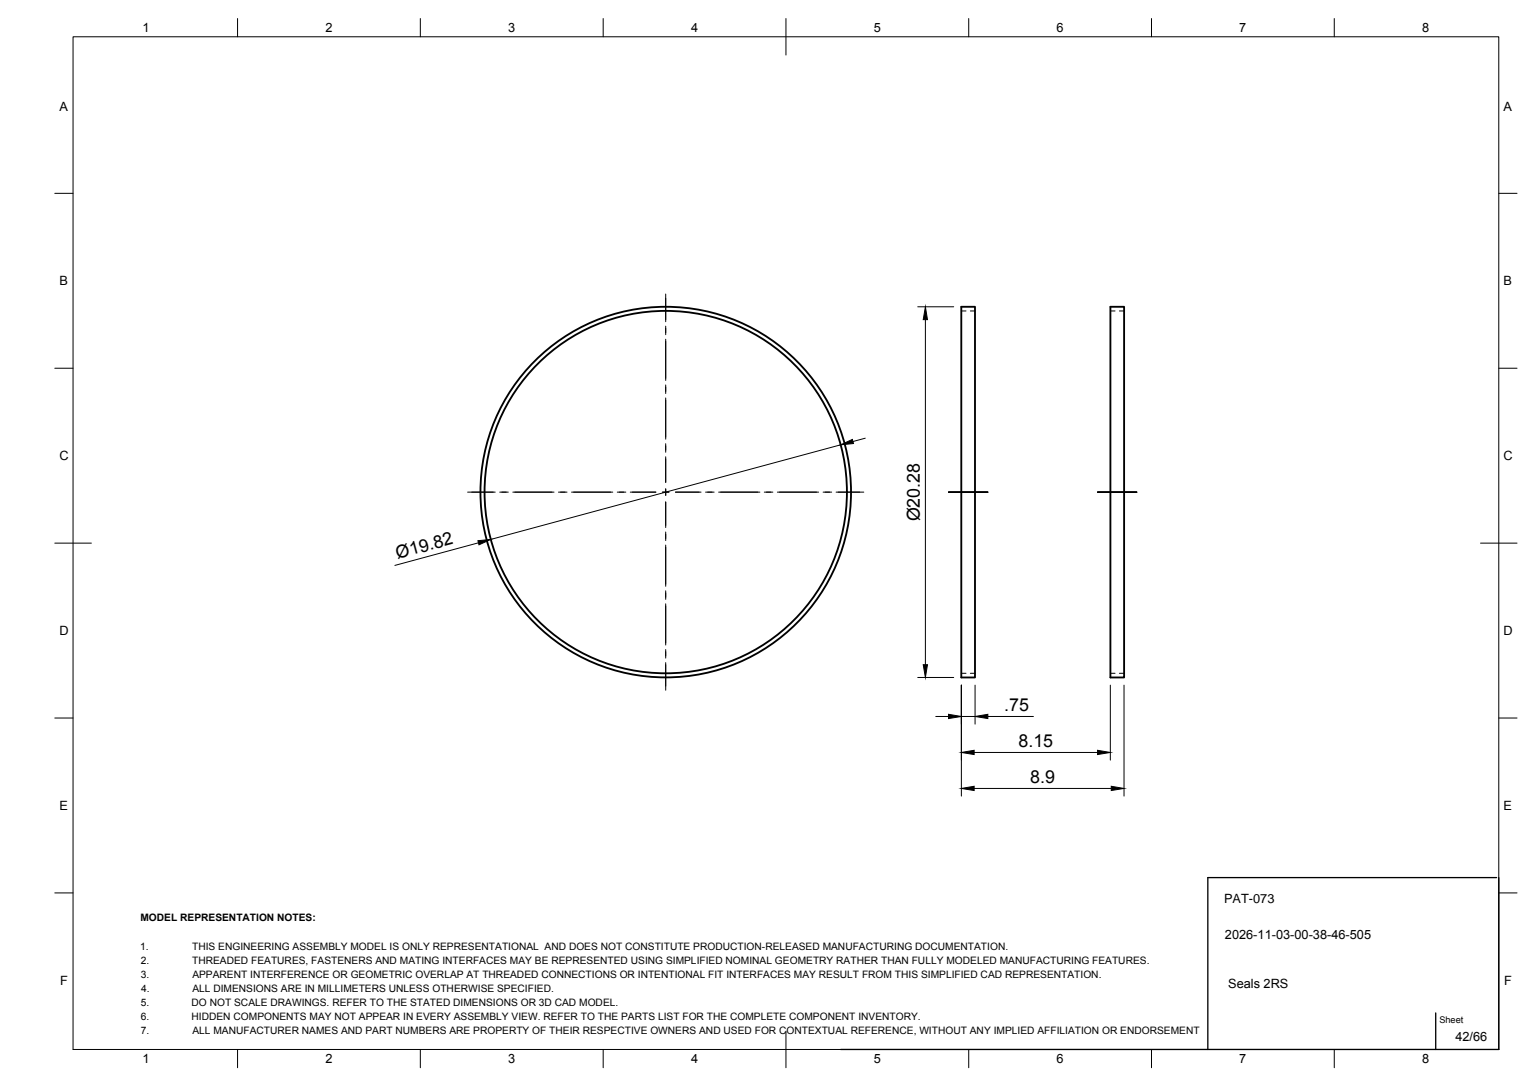
ISO-10303-21;
HEADER;
/* Generated by software containing ST-Developer
 * from STEP Tools, Inc. (www.steptools.com) 
 */

FILE_DESCRIPTION(
/* description */ ('Manual piston pump'),
/* implementation_level */ '2;1');

FILE_NAME(
/* name */ 'Seals 2RS.step',
/* time_stamp */ '2026-11-02T16:54:23-08:00',
/* author */ (''),
/* organization */ (''),
/* preprocessor_version */ 'ST-DEVELOPER v20.2',
/* originating_system */ 'Autodesk Translation Framework v15.17.0.0',
/* authorisation */ '');

FILE_SCHEMA (('AUTOMOTIVE_DESIGN { 1 0 10303 214 3 1 1 }'));
ENDSEC;

DATA;
#10=MECHANICAL_DESIGN_GEOMETRIC_PRESENTATION_REPRESENTATION('',(#722,#723),#19043);
#589=SHAPE_REPRESENTATION_RELATIONSHIP('SRR','None',#19336,#652);
#652=ADVANCED_BREP_SHAPE_REPRESENTATION('',(#792,#793),#19003);
#722=STYLED_ITEM('',(#19661),#792);
#723=STYLED_ITEM('',(#19661),#793);
#792=MANIFOLD_SOLID_BREP('Body1',#9508);
#793=MANIFOLD_SOLID_BREP('Body2',#9509);
#951=FACE_BOUND('',#2273,.T.);
#952=FACE_BOUND('',#2276,.T.);
#953=FACE_BOUND('',#2279,.T.);
#954=FACE_BOUND('',#2282,.T.);
#1191=CYLINDRICAL_SURFACE('',#10820,1.013815);
#1192=CYLINDRICAL_SURFACE('',#10824,0.991185);
#1193=CYLINDRICAL_SURFACE('',#10828,1.013815);
#1194=CYLINDRICAL_SURFACE('',#10832,0.991185);
#1573=FACE_OUTER_BOUND('',#2272,.T.);
#1574=FACE_OUTER_BOUND('',#2274,.T.);
#1575=FACE_OUTER_BOUND('',#2275,.T.);
#1576=FACE_OUTER_BOUND('',#2277,.T.);
#1577=FACE_OUTER_BOUND('',#2278,.T.);
#1578=FACE_OUTER_BOUND('',#2280,.T.);
#1579=FACE_OUTER_BOUND('',#2281,.T.);
#1580=FACE_OUTER_BOUND('',#2283,.T.);
#2272=EDGE_LOOP('',(#7437));
#2273=EDGE_LOOP('',(#7438));
#2274=EDGE_LOOP('',(#7439,#7440,#7441,#7442));
#2275=EDGE_LOOP('',(#7443));
#2276=EDGE_LOOP('',(#7444));
#2277=EDGE_LOOP('',(#7445,#7446,#7447,#7448));
#2278=EDGE_LOOP('',(#7449));
#2279=EDGE_LOOP('',(#7450));
#2280=EDGE_LOOP('',(#7451,#7452,#7453,#7454));
#2281=EDGE_LOOP('',(#7455));
#2282=EDGE_LOOP('',(#7456));
#2283=EDGE_LOOP('',(#7457,#7458,#7459,#7460));
#2925=CIRCLE('',#10818,1.013815);
#2926=CIRCLE('',#10819,0.991185);
#2927=CIRCLE('',#10821,1.013815);
#2928=CIRCLE('',#10823,0.991185);
#2929=CIRCLE('',#10826,1.013815);
#2930=CIRCLE('',#10827,0.991185);
#2931=CIRCLE('',#10829,1.013815);
#2932=CIRCLE('',#10831,0.991185);
#3434=LINE('',#16311,#4038);
#3435=LINE('',#16316,#4039);
#3436=LINE('',#16325,#4040);
#3437=LINE('',#16330,#4041);
#4038=VECTOR('',#12940,1.013815);
#4039=VECTOR('',#12947,0.991185);
#4040=VECTOR('',#12958,1.013815);
#4041=VECTOR('',#12965,0.991185);
#4748=VERTEX_POINT('',#16304);
#4749=VERTEX_POINT('',#16306);
#4750=VERTEX_POINT('',#16309);
#4751=VERTEX_POINT('',#16313);
#4752=VERTEX_POINT('',#16318);
#4753=VERTEX_POINT('',#16320);
#4754=VERTEX_POINT('',#16323);
#4755=VERTEX_POINT('',#16327);
#5705=EDGE_CURVE('',#4748,#4748,#2925,.T.);
#5706=EDGE_CURVE('',#4749,#4749,#2926,.T.);
#5707=EDGE_CURVE('',#4750,#4750,#2927,.T.);
#5708=EDGE_CURVE('',#4750,#4748,#3434,.T.);
#5709=EDGE_CURVE('',#4751,#4751,#2928,.T.);
#5710=EDGE_CURVE('',#4751,#4749,#3435,.T.);
#5711=EDGE_CURVE('',#4752,#4752,#2929,.T.);
#5712=EDGE_CURVE('',#4753,#4753,#2930,.T.);
#5713=EDGE_CURVE('',#4754,#4754,#2931,.T.);
#5714=EDGE_CURVE('',#4754,#4752,#3436,.T.);
#5715=EDGE_CURVE('',#4755,#4755,#2932,.T.);
#5716=EDGE_CURVE('',#4755,#4753,#3437,.T.);
#7437=ORIENTED_EDGE('',*,*,#5705,.F.);
#7438=ORIENTED_EDGE('',*,*,#5706,.T.);
#7439=ORIENTED_EDGE('',*,*,#5707,.F.);
#7440=ORIENTED_EDGE('',*,*,#5708,.T.);
#7441=ORIENTED_EDGE('',*,*,#5705,.T.);
#7442=ORIENTED_EDGE('',*,*,#5708,.F.);
#7443=ORIENTED_EDGE('',*,*,#5707,.T.);
#7444=ORIENTED_EDGE('',*,*,#5709,.F.);
#7445=ORIENTED_EDGE('',*,*,#5709,.T.);
#7446=ORIENTED_EDGE('',*,*,#5710,.T.);
#7447=ORIENTED_EDGE('',*,*,#5706,.F.);
#7448=ORIENTED_EDGE('',*,*,#5710,.F.);
#7449=ORIENTED_EDGE('',*,*,#5711,.F.);
#7450=ORIENTED_EDGE('',*,*,#5712,.T.);
#7451=ORIENTED_EDGE('',*,*,#5713,.F.);
#7452=ORIENTED_EDGE('',*,*,#5714,.T.);
#7453=ORIENTED_EDGE('',*,*,#5711,.T.);
#7454=ORIENTED_EDGE('',*,*,#5714,.F.);
#7455=ORIENTED_EDGE('',*,*,#5713,.T.);
#7456=ORIENTED_EDGE('',*,*,#5715,.F.);
#7457=ORIENTED_EDGE('',*,*,#5715,.T.);
#7458=ORIENTED_EDGE('',*,*,#5716,.T.);
#7459=ORIENTED_EDGE('',*,*,#5712,.F.);
#7460=ORIENTED_EDGE('',*,*,#5716,.F.);
#8721=PLANE('',#10817);
#8722=PLANE('',#10822);
#8723=PLANE('',#10825);
#8724=PLANE('',#10830);
#9178=ADVANCED_FACE('',(#1573,#951),#8721,.T.);
#9179=ADVANCED_FACE('',(#1574),#1191,.T.);
#9180=ADVANCED_FACE('',(#1575,#952),#8722,.T.);
#9181=ADVANCED_FACE('',(#1576),#1192,.F.);
#9182=ADVANCED_FACE('',(#1577,#953),#8723,.T.);
#9183=ADVANCED_FACE('',(#1578),#1193,.T.);
#9184=ADVANCED_FACE('',(#1579,#954),#8724,.T.);
#9185=ADVANCED_FACE('',(#1580),#1194,.F.);
#9508=CLOSED_SHELL('',(#9178,#9179,#9180,#9181));
#9509=CLOSED_SHELL('',(#9182,#9183,#9184,#9185));
#10816=AXIS2_PLACEMENT_3D('',#16302,#12928,#12929);
#10817=AXIS2_PLACEMENT_3D('',#16303,#12930,#12931);
#10818=AXIS2_PLACEMENT_3D('',#16305,#12932,#12933);
#10819=AXIS2_PLACEMENT_3D('',#16307,#12934,#12935);
#10820=AXIS2_PLACEMENT_3D('',#16308,#12936,#12937);
#10821=AXIS2_PLACEMENT_3D('',#16310,#12938,#12939);
#10822=AXIS2_PLACEMENT_3D('',#16312,#12941,#12942);
#10823=AXIS2_PLACEMENT_3D('',#16314,#12943,#12944);
#10824=AXIS2_PLACEMENT_3D('',#16315,#12945,#12946);
#10825=AXIS2_PLACEMENT_3D('',#16317,#12948,#12949);
#10826=AXIS2_PLACEMENT_3D('',#16319,#12950,#12951);
#10827=AXIS2_PLACEMENT_3D('',#16321,#12952,#12953);
#10828=AXIS2_PLACEMENT_3D('',#16322,#12954,#12955);
#10829=AXIS2_PLACEMENT_3D('',#16324,#12956,#12957);
#10830=AXIS2_PLACEMENT_3D('',#16326,#12959,#12960);
#10831=AXIS2_PLACEMENT_3D('',#16328,#12961,#12962);
#10832=AXIS2_PLACEMENT_3D('',#16329,#12963,#12964);
#12928=DIRECTION('axis',(0.,0.,1.));
#12929=DIRECTION('refdir',(1.,0.,0.));
#12930=DIRECTION('center_axis',(0.,1.,0.));
#12931=DIRECTION('ref_axis',(0.,0.,1.));
#12932=DIRECTION('center_axis',(0.,-1.,0.));
#12933=DIRECTION('ref_axis',(1.,0.,0.));
#12934=DIRECTION('center_axis',(0.,-1.,0.));
#12935=DIRECTION('ref_axis',(1.,0.,0.));
#12936=DIRECTION('center_axis',(0.,-1.,0.));
#12937=DIRECTION('ref_axis',(1.,0.,0.));
#12938=DIRECTION('center_axis',(0.,-1.,0.));
#12939=DIRECTION('ref_axis',(1.,0.,0.));
#12940=DIRECTION('',(0.,1.,0.));
#12941=DIRECTION('center_axis',(0.,-1.,0.));
#12942=DIRECTION('ref_axis',(0.,0.,-1.));
#12943=DIRECTION('center_axis',(0.,-1.,0.));
#12944=DIRECTION('ref_axis',(1.,0.,0.));
#12945=DIRECTION('center_axis',(0.,-1.,0.));
#12946=DIRECTION('ref_axis',(1.,0.,0.));
#12947=DIRECTION('',(0.,1.,0.));
#12948=DIRECTION('center_axis',(0.,1.,0.));
#12949=DIRECTION('ref_axis',(0.,0.,1.));
#12950=DIRECTION('center_axis',(0.,-1.,0.));
#12951=DIRECTION('ref_axis',(1.,0.,0.));
#12952=DIRECTION('center_axis',(0.,-1.,0.));
#12953=DIRECTION('ref_axis',(1.,0.,0.));
#12954=DIRECTION('center_axis',(0.,-1.,0.));
#12955=DIRECTION('ref_axis',(1.,0.,0.));
#12956=DIRECTION('center_axis',(0.,-1.,0.));
#12957=DIRECTION('ref_axis',(1.,0.,0.));
#12958=DIRECTION('',(0.,1.,0.));
#12959=DIRECTION('center_axis',(0.,-1.,0.));
#12960=DIRECTION('ref_axis',(0.,0.,-1.));
#12961=DIRECTION('center_axis',(0.,-1.,0.));
#12962=DIRECTION('ref_axis',(1.,0.,0.));
#12963=DIRECTION('center_axis',(0.,-1.,0.));
#12964=DIRECTION('ref_axis',(1.,0.,0.));
#12965=DIRECTION('',(0.,1.,0.));
#16302=CARTESIAN_POINT('',(0.,0.,0.));
#16303=CARTESIAN_POINT('Origin',(1.013815,0.445,0.));
#16304=CARTESIAN_POINT('',(-1.013815,0.445,-1.24156529467757E-16));
#16305=CARTESIAN_POINT('Origin',(0.,0.445,0.));
#16306=CARTESIAN_POINT('',(-0.991185,0.445,-1.21385153761287E-16));
#16307=CARTESIAN_POINT('Origin',(0.,0.445,0.));
#16308=CARTESIAN_POINT('Origin',(0.,0.4075,0.));
#16309=CARTESIAN_POINT('',(-1.013815,0.37,-1.24156529467757E-16));
#16310=CARTESIAN_POINT('Origin',(0.,0.37,0.));
#16311=CARTESIAN_POINT('',(-1.013815,0.4075,-1.24156529467757E-16));
#16312=CARTESIAN_POINT('Origin',(0.991185,0.37,0.));
#16313=CARTESIAN_POINT('',(-0.991185,0.37,-1.21385153761287E-16));
#16314=CARTESIAN_POINT('Origin',(0.,0.37,0.));
#16315=CARTESIAN_POINT('Origin',(0.,0.4075,0.));
#16316=CARTESIAN_POINT('',(-0.991185,0.4075,-1.21385153761287E-16));
#16317=CARTESIAN_POINT('Origin',(1.013815,-0.37,0.));
#16318=CARTESIAN_POINT('',(-1.013815,-0.37,-1.24156529467757E-16));
#16319=CARTESIAN_POINT('Origin',(0.,-0.37,0.));
#16320=CARTESIAN_POINT('',(-0.991185,-0.37,-1.21385153761287E-16));
#16321=CARTESIAN_POINT('Origin',(0.,-0.37,0.));
#16322=CARTESIAN_POINT('Origin',(0.,-0.4075,0.));
#16323=CARTESIAN_POINT('',(-1.013815,-0.445,-1.24156529467757E-16));
#16324=CARTESIAN_POINT('Origin',(0.,-0.445,0.));
#16325=CARTESIAN_POINT('',(-1.013815,-0.4075,-1.24156529467757E-16));
#16326=CARTESIAN_POINT('Origin',(0.991185,-0.445,0.));
#16327=CARTESIAN_POINT('',(-0.991185,-0.445,-1.21385153761287E-16));
#16328=CARTESIAN_POINT('Origin',(0.,-0.445,0.));
#16329=CARTESIAN_POINT('Origin',(0.,-0.4075,0.));
#16330=CARTESIAN_POINT('',(-0.991185,-0.4075,-1.21385153761287E-16));
#18932=UNCERTAINTY_MEASURE_WITH_UNIT(LENGTH_MEASURE(0.001),#19044,
'DISTANCE_ACCURACY_VALUE',
'Maximum model space distance between geometric entities at asserted c
onnectivities');
#18972=UNCERTAINTY_MEASURE_WITH_UNIT(LENGTH_MEASURE(0.001),#19044,
'DISTANCE_ACCURACY_VALUE',
'Maximum model space distance between geometric entities at asserted c
onnectivities');
#19003=(
GEOMETRIC_REPRESENTATION_CONTEXT(3)
GLOBAL_UNCERTAINTY_ASSIGNED_CONTEXT((#18932))
GLOBAL_UNIT_ASSIGNED_CONTEXT((#19044,#19046,#19047))
REPRESENTATION_CONTEXT('','3D')
);
#19043=(
GEOMETRIC_REPRESENTATION_CONTEXT(3)
GLOBAL_UNCERTAINTY_ASSIGNED_CONTEXT((#18972))
GLOBAL_UNIT_ASSIGNED_CONTEXT((#19044,#19046,#19047))
REPRESENTATION_CONTEXT('','3D')
);
#19044=(
LENGTH_UNIT()
NAMED_UNIT(*)
SI_UNIT(.CENTI.,.METRE.)
);
#19046=(
NAMED_UNIT(*)
PLANE_ANGLE_UNIT()
SI_UNIT($,.RADIAN.)
);
#19047=(
NAMED_UNIT(*)
SI_UNIT($,.STERADIAN.)
SOLID_ANGLE_UNIT()
);
#19078=SHAPE_DEFINITION_REPRESENTATION(#19148,#19336);
#19148=PRODUCT_DEFINITION_SHAPE('',$,#19407);
#19336=SHAPE_REPRESENTATION('',(#10816),#19003);
#19376=PRODUCT_DEFINITION_CONTEXT('part definition',#19588,'design');
#19407=PRODUCT_DEFINITION('2026-11-03-00-38-46-505','Seals 2RS',#19477,
#19376);
#19477=PRODUCT_DEFINITION_FORMATION('',$,#19620);
#19588=APPLICATION_CONTEXT(
'Core Data for Automotive Mechanical Design Process');
#19589=PRODUCT_CONTEXT('part definition',#19588,'mechanical');
#19620=PRODUCT('2026-11-03-00-38-46-505','Seals 2RS','Seals 2RS',(#19589));
#19661=PRESENTATION_STYLE_ASSIGNMENT((#19667));
#19667=SURFACE_STYLE_USAGE(.BOTH.,#19673);
#19673=SURFACE_SIDE_STYLE('',(#19679));
#19679=SURFACE_STYLE_FILL_AREA(#19685);
#19685=FILL_AREA_STYLE('CAD Library Painted - Engineering blue',(#19691));
#19691=FILL_AREA_STYLE_COLOUR('CAD Library Painted - Engineering blue',
#19697);
#19697=COLOUR_RGB('CAD Library Painted - Engineering blue',0.12156862745098,
0.356862745098039,0.6);
ENDSEC;
END-ISO-10303-21;
